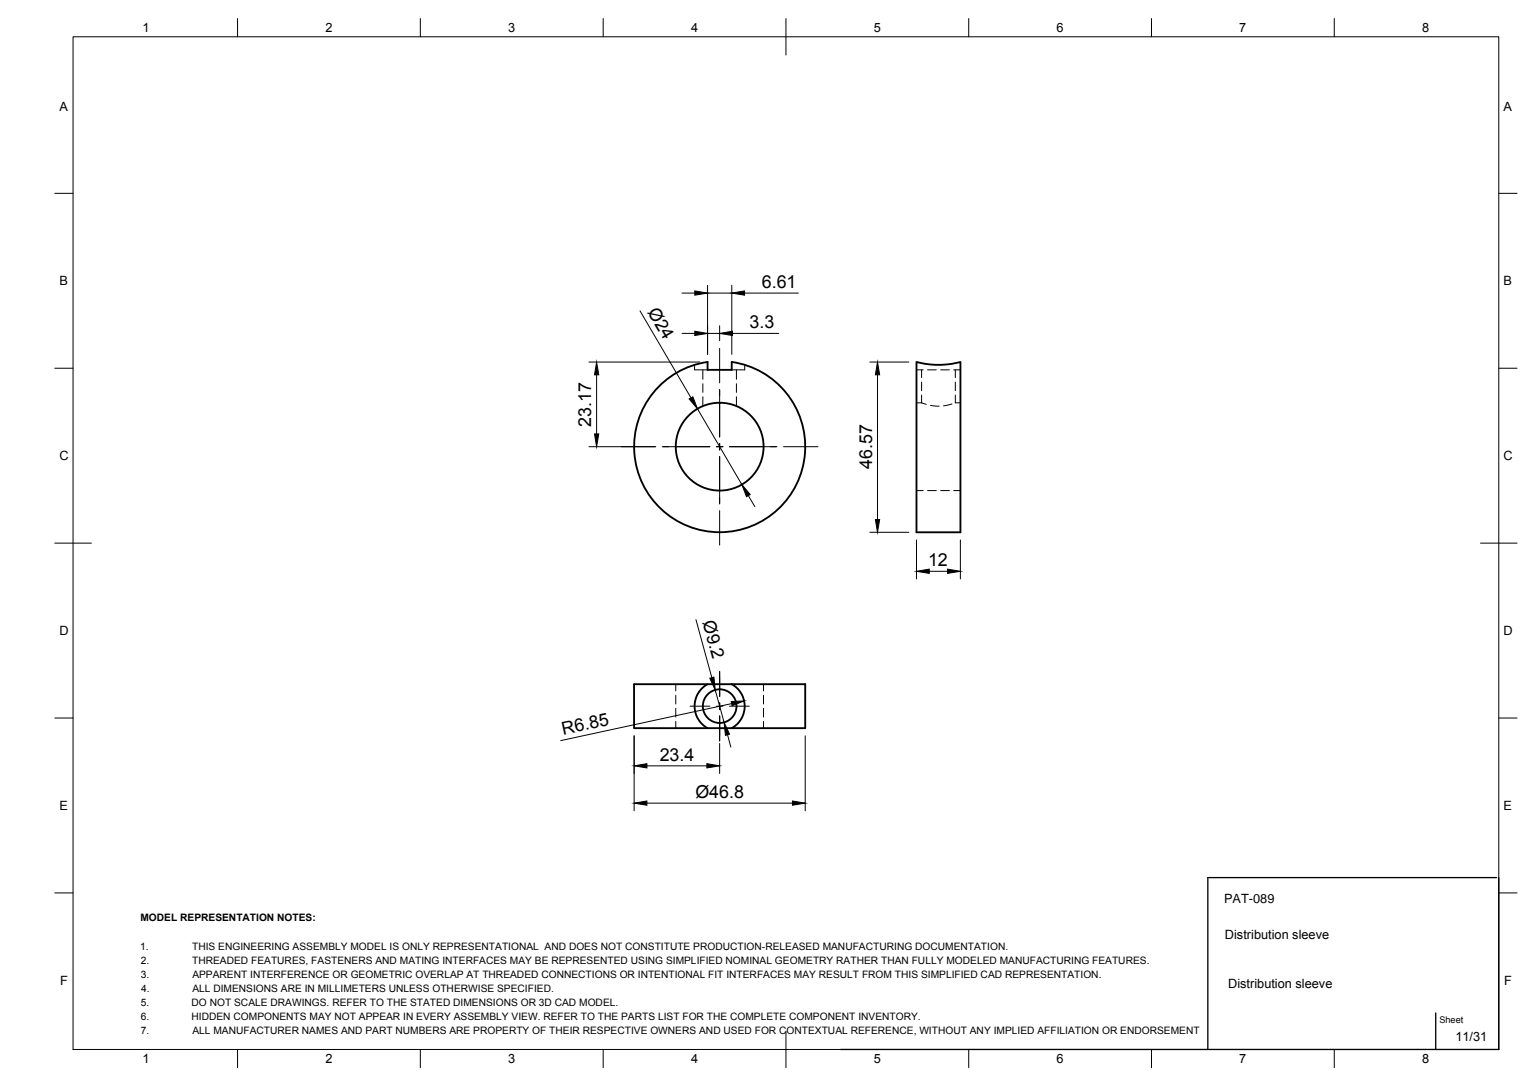
ISO-10303-21;
HEADER;
/* Generated by software containing ST-Developer
 * from STEP Tools, Inc. (www.steptools.com) 
 */

FILE_DESCRIPTION(
/* description */ ('Rotary union on bearing shaft'),
/* implementation_level */ '2;1');

FILE_NAME(
/* name */ 'Distribution sleeve.step',
/* time_stamp */ '2026-10-28T03:24:01-07:00',
/* author */ (''),
/* organization */ (''),
/* preprocessor_version */ 'ST-DEVELOPER v20.2',
/* originating_system */ 'Autodesk Translation Framework v15.17.0.0',
/* authorisation */ '');

FILE_SCHEMA (('AUTOMOTIVE_DESIGN { 1 0 10303 214 3 1 1 }'));
ENDSEC;

DATA;
#10=MECHANICAL_DESIGN_GEOMETRIC_PRESENTATION_REPRESENTATION('',(#319),#9448);
#229=B_SPLINE_CURVE_WITH_KNOTS('',3,(#7786,#7787,#7788,#7789,#7790,#7791,
#7792,#7793,#7794,#7795,#7796,#7797,#7798,#7799,#7800),.UNSPECIFIED.,.F.,
 .F.,(4,2,2,3,2,2,4),(-0.70773137284392,-0.519428793117576,-0.259714396558788,
0.,0.259714396558788,0.519428793117576,0.707731372984028),.UNSPECIFIED.);
#230=B_SPLINE_CURVE_WITH_KNOTS('',3,(#7812,#7813,#7814,#7815,#7816,#7817,
#7818,#7819,#7820,#7821,#7822,#7823,#7824,#7825),.UNSPECIFIED.,.F.,.F.,
(4,2,2,2,2,2,4),(1.36970442594422,1.55800700581067,1.81772140236946,2.07743579892825,
2.33715019548703,2.59686459204582,2.78516717191228),.UNSPECIFIED.);
#231=B_SPLINE_CURVE_WITH_KNOTS('',3,(#7840,#7841,#7842,#7843,#7844,#7845,
#7846,#7847,#7848,#7849,#7850,#7851,#7852,#7853,#7854,#7855,#7856,#7857),
 .UNSPECIFIED.,.F.,.F.,(4,2,2,2,2,2,2,2,4),(0.,0.175311710953118,0.350623421906236,
0.525787580035871,0.700951738165507,0.876115896295143,1.05128005442478,
1.2265917653779,1.40190347633101),.UNSPECIFIED.);
#232=B_SPLINE_CURVE_WITH_KNOTS('',3,(#7858,#7859,#7860,#7861,#7862,#7863,
#7864,#7865,#7866,#7867,#7868,#7869,#7870,#7871,#7872,#7873,#7874,#7875),
 .UNSPECIFIED.,.F.,.F.,(4,2,2,2,2,2,2,2,4),(1.40190347633101,1.57721518728413,
1.75252689823725,1.92769105636689,2.10285521449652,2.27801937262616,2.45318353075579,
2.62849524170891,2.80380695266203),.UNSPECIFIED.);
#265=SHAPE_REPRESENTATION_RELATIONSHIP('SRR','None',#9565,#292);
#292=ADVANCED_BREP_SHAPE_REPRESENTATION('',(#354),#9425);
#319=STYLED_ITEM('',(#9764),#354);
#354=MANIFOLD_SOLID_BREP('Body1',#4874);
#418=FACE_BOUND('',#1067,.T.);
#419=FACE_BOUND('',#1069,.T.);
#420=FACE_BOUND('',#1073,.T.);
#421=FACE_BOUND('',#1075,.T.);
#529=PLANE('',#5352);
#530=PLANE('',#5354);
#531=PLANE('',#5362);
#727=FACE_OUTER_BOUND('',#1064,.T.);
#728=FACE_OUTER_BOUND('',#1065,.T.);
#729=FACE_OUTER_BOUND('',#1066,.T.);
#730=FACE_OUTER_BOUND('',#1068,.T.);
#731=FACE_OUTER_BOUND('',#1070,.T.);
#732=FACE_OUTER_BOUND('',#1071,.T.);
#733=FACE_OUTER_BOUND('',#1072,.T.);
#734=FACE_OUTER_BOUND('',#1074,.T.);
#1064=EDGE_LOOP('',(#3553,#3554,#3555,#3556));
#1065=EDGE_LOOP('',(#3557,#3558,#3559,#3560));
#1066=EDGE_LOOP('',(#3561,#3562,#3563,#3564));
#1067=EDGE_LOOP('',(#3565));
#1068=EDGE_LOOP('',(#3566,#3567,#3568,#3569));
#1069=EDGE_LOOP('',(#3570));
#1070=EDGE_LOOP('',(#3571,#3572,#3573,#3574));
#1071=EDGE_LOOP('',(#3575,#3576,#3577,#3578,#3579));
#1072=EDGE_LOOP('',(#3580,#3581,#3582,#3583));
#1073=EDGE_LOOP('',(#3584,#3585));
#1074=EDGE_LOOP('',(#3586,#3587,#3588,#3589));
#1075=EDGE_LOOP('',(#3590));
#1436=LINE('',#7784,#1756);
#1437=LINE('',#7802,#1757);
#1438=LINE('',#7807,#1758);
#1439=LINE('',#7811,#1759);
#1440=LINE('',#7827,#1760);
#1441=LINE('',#7828,#1761);
#1442=LINE('',#7876,#1762);
#1443=LINE('',#7879,#1763);
#1756=VECTOR('',#6193,1.);
#1757=VECTOR('',#6194,1.);
#1758=VECTOR('',#6199,1.);
#1759=VECTOR('',#6202,1.);
#1760=VECTOR('',#6205,1.);
#1761=VECTOR('',#6206,1.);
#1762=VECTOR('',#6221,0.46);
#1763=VECTOR('',#6224,1.2);
#2065=CIRCLE('',#5349,0.685);
#2066=CIRCLE('',#5351,0.685);
#2067=CIRCLE('',#5353,0.46);
#2068=CIRCLE('',#5355,2.34);
#2069=CIRCLE('',#5356,1.2);
#2070=CIRCLE('',#5358,2.34);
#2071=CIRCLE('',#5361,1.2);
#2347=VERTEX_POINT('',#7782);
#2348=VERTEX_POINT('',#7783);
#2349=VERTEX_POINT('',#7785);
#2350=VERTEX_POINT('',#7801);
#2351=VERTEX_POINT('',#7805);
#2352=VERTEX_POINT('',#7806);
#2353=VERTEX_POINT('',#7808);
#2354=VERTEX_POINT('',#7810);
#2355=VERTEX_POINT('',#7829);
#2356=VERTEX_POINT('',#7833);
#2357=VERTEX_POINT('',#7838);
#2358=VERTEX_POINT('',#7839);
#2359=VERTEX_POINT('',#7878);
#2804=EDGE_CURVE('',#2347,#2348,#1436,.T.);
#2805=EDGE_CURVE('',#2349,#2347,#229,.T.);
#2806=EDGE_CURVE('',#2350,#2349,#1437,.T.);
#2807=EDGE_CURVE('',#2348,#2350,#2065,.T.);
#2808=EDGE_CURVE('',#2351,#2352,#1438,.T.);
#2809=EDGE_CURVE('',#2353,#2351,#2066,.T.);
#2810=EDGE_CURVE('',#2354,#2353,#1439,.T.);
#2811=EDGE_CURVE('',#2352,#2354,#230,.T.);
#2812=EDGE_CURVE('',#2348,#2351,#1440,.T.);
#2813=EDGE_CURVE('',#2353,#2350,#1441,.T.);
#2814=EDGE_CURVE('',#2355,#2355,#2067,.T.);
#2815=EDGE_CURVE('',#2349,#2354,#2068,.T.);
#2816=EDGE_CURVE('',#2356,#2356,#2069,.T.);
#2817=EDGE_CURVE('',#2347,#2352,#2070,.T.);
#2818=EDGE_CURVE('',#2357,#2358,#231,.T.);
#2819=EDGE_CURVE('',#2358,#2357,#232,.T.);
#2820=EDGE_CURVE('',#2358,#2355,#1442,.T.);
#2821=EDGE_CURVE('',#2356,#2359,#1443,.T.);
#2822=EDGE_CURVE('',#2359,#2359,#2071,.T.);
#3553=ORIENTED_EDGE('',*,*,#2804,.F.);
#3554=ORIENTED_EDGE('',*,*,#2805,.F.);
#3555=ORIENTED_EDGE('',*,*,#2806,.F.);
#3556=ORIENTED_EDGE('',*,*,#2807,.F.);
#3557=ORIENTED_EDGE('',*,*,#2808,.F.);
#3558=ORIENTED_EDGE('',*,*,#2809,.F.);
#3559=ORIENTED_EDGE('',*,*,#2810,.F.);
#3560=ORIENTED_EDGE('',*,*,#2811,.F.);
#3561=ORIENTED_EDGE('',*,*,#2812,.F.);
#3562=ORIENTED_EDGE('',*,*,#2807,.T.);
#3563=ORIENTED_EDGE('',*,*,#2813,.F.);
#3564=ORIENTED_EDGE('',*,*,#2809,.T.);
#3565=ORIENTED_EDGE('',*,*,#2814,.F.);
#3566=ORIENTED_EDGE('',*,*,#2810,.T.);
#3567=ORIENTED_EDGE('',*,*,#2813,.T.);
#3568=ORIENTED_EDGE('',*,*,#2806,.T.);
#3569=ORIENTED_EDGE('',*,*,#2815,.T.);
#3570=ORIENTED_EDGE('',*,*,#2816,.T.);
#3571=ORIENTED_EDGE('',*,*,#2811,.T.);
#3572=ORIENTED_EDGE('',*,*,#2815,.F.);
#3573=ORIENTED_EDGE('',*,*,#2805,.T.);
#3574=ORIENTED_EDGE('',*,*,#2817,.T.);
#3575=ORIENTED_EDGE('',*,*,#2818,.F.);
#3576=ORIENTED_EDGE('',*,*,#2819,.F.);
#3577=ORIENTED_EDGE('',*,*,#2820,.T.);
#3578=ORIENTED_EDGE('',*,*,#2814,.T.);
#3579=ORIENTED_EDGE('',*,*,#2820,.F.);
#3580=ORIENTED_EDGE('',*,*,#2816,.F.);
#3581=ORIENTED_EDGE('',*,*,#2821,.T.);
#3582=ORIENTED_EDGE('',*,*,#2822,.T.);
#3583=ORIENTED_EDGE('',*,*,#2821,.F.);
#3584=ORIENTED_EDGE('',*,*,#2818,.T.);
#3585=ORIENTED_EDGE('',*,*,#2819,.T.);
#3586=ORIENTED_EDGE('',*,*,#2808,.T.);
#3587=ORIENTED_EDGE('',*,*,#2817,.F.);
#3588=ORIENTED_EDGE('',*,*,#2804,.T.);
#3589=ORIENTED_EDGE('',*,*,#2812,.T.);
#3590=ORIENTED_EDGE('',*,*,#2822,.F.);
#4506=CYLINDRICAL_SURFACE('',#5348,0.685);
#4507=CYLINDRICAL_SURFACE('',#5350,0.685);
#4508=CYLINDRICAL_SURFACE('',#5357,2.34);
#4509=CYLINDRICAL_SURFACE('',#5359,0.46);
#4510=CYLINDRICAL_SURFACE('',#5360,1.2);
#4640=ADVANCED_FACE('',(#727),#4506,.F.);
#4641=ADVANCED_FACE('',(#728),#4507,.F.);
#4642=ADVANCED_FACE('',(#729,#418),#529,.T.);
#4643=ADVANCED_FACE('',(#730,#419),#530,.T.);
#4644=ADVANCED_FACE('',(#731),#4508,.T.);
#4645=ADVANCED_FACE('',(#732),#4509,.F.);
#4646=ADVANCED_FACE('',(#733,#420),#4510,.F.);
#4647=ADVANCED_FACE('',(#734,#421),#531,.F.);
#4874=CLOSED_SHELL('',(#4640,#4641,#4642,#4643,#4644,#4645,#4646,#4647));
#5347=AXIS2_PLACEMENT_3D('',#7780,#6189,#6190);
#5348=AXIS2_PLACEMENT_3D('',#7781,#6191,#6192);
#5349=AXIS2_PLACEMENT_3D('',#7803,#6195,#6196);
#5350=AXIS2_PLACEMENT_3D('',#7804,#6197,#6198);
#5351=AXIS2_PLACEMENT_3D('',#7809,#6200,#6201);
#5352=AXIS2_PLACEMENT_3D('',#7826,#6203,#6204);
#5353=AXIS2_PLACEMENT_3D('',#7830,#6207,#6208);
#5354=AXIS2_PLACEMENT_3D('',#7831,#6209,#6210);
#5355=AXIS2_PLACEMENT_3D('',#7832,#6211,#6212);
#5356=AXIS2_PLACEMENT_3D('',#7834,#6213,#6214);
#5357=AXIS2_PLACEMENT_3D('',#7835,#6215,#6216);
#5358=AXIS2_PLACEMENT_3D('',#7836,#6217,#6218);
#5359=AXIS2_PLACEMENT_3D('',#7837,#6219,#6220);
#5360=AXIS2_PLACEMENT_3D('',#7877,#6222,#6223);
#5361=AXIS2_PLACEMENT_3D('',#7880,#6225,#6226);
#5362=AXIS2_PLACEMENT_3D('',#7881,#6227,#6228);
#6189=DIRECTION('axis',(0.,0.,1.));
#6190=DIRECTION('refdir',(1.,0.,0.));
#6191=DIRECTION('center_axis',(1.,0.,0.));
#6192=DIRECTION('ref_axis',(0.,0.,-1.));
#6193=DIRECTION('',(-1.,0.,0.));
#6194=DIRECTION('',(1.,0.,0.));
#6195=DIRECTION('center_axis',(1.,0.,0.));
#6196=DIRECTION('ref_axis',(0.,0.,-1.));
#6197=DIRECTION('center_axis',(1.,0.,0.));
#6198=DIRECTION('ref_axis',(0.,7.6571373978539E-16,1.));
#6199=DIRECTION('',(1.,0.,0.));
#6200=DIRECTION('center_axis',(1.,0.,0.));
#6201=DIRECTION('ref_axis',(0.,0.,-1.));
#6202=DIRECTION('',(-1.,0.,0.));
#6203=DIRECTION('center_axis',(1.,0.,0.));
#6204=DIRECTION('ref_axis',(0.,0.,-1.));
#6205=DIRECTION('',(0.,0.,1.));
#6206=DIRECTION('',(0.,0.,-1.));
#6207=DIRECTION('center_axis',(1.,0.,0.));
#6208=DIRECTION('ref_axis',(0.,0.,-1.));
#6209=DIRECTION('center_axis',(0.,1.,0.));
#6210=DIRECTION('ref_axis',(1.,0.,0.));
#6211=DIRECTION('center_axis',(0.,1.,0.));
#6212=DIRECTION('ref_axis',(1.,0.,0.));
#6213=DIRECTION('center_axis',(0.,-1.,0.));
#6214=DIRECTION('ref_axis',(1.,0.,0.));
#6215=DIRECTION('center_axis',(0.,1.,0.));
#6216=DIRECTION('ref_axis',(-1.,0.,1.22464679914735E-16));
#6217=DIRECTION('center_axis',(0.,1.,0.));
#6218=DIRECTION('ref_axis',(1.,0.,0.));
#6219=DIRECTION('center_axis',(1.,0.,0.));
#6220=DIRECTION('ref_axis',(0.,0.,-1.));
#6221=DIRECTION('',(1.,0.,0.));
#6222=DIRECTION('center_axis',(0.,1.,0.));
#6223=DIRECTION('ref_axis',(1.,0.,0.));
#6224=DIRECTION('',(0.,-1.,0.));
#6225=DIRECTION('center_axis',(0.,-1.,0.));
#6226=DIRECTION('ref_axis',(1.,0.,0.));
#6227=DIRECTION('center_axis',(0.,1.,0.));
#6228=DIRECTION('ref_axis',(1.,0.,0.));
#7780=CARTESIAN_POINT('',(0.,0.,0.));
#7781=CARTESIAN_POINT('Origin',(2.1,3.,4.5));
#7782=CARTESIAN_POINT('',(2.3165437617278,2.4,4.16950794260678));
#7783=CARTESIAN_POINT('',(2.1,2.4,4.16950794260678));
#7784=CARTESIAN_POINT('',(2.1,2.4,4.16950794260678));
#7785=CARTESIAN_POINT('',(2.3165437617278,3.6,4.16950794260679));
#7786=CARTESIAN_POINT('Ctrl Pts',(2.3165437617278,3.6,4.16950794260679));
#7787=CARTESIAN_POINT('Ctrl Pts',(2.30831151031136,3.56821604889379,4.11180498050191));
#7788=CARTESIAN_POINT('Ctrl Pts',(2.29860746123388,3.52826296991183,4.05952667968626));
#7789=CARTESIAN_POINT('Ctrl Pts',(2.27651111163957,3.42382665942891,3.95509036920334));
#7790=CARTESIAN_POINT('Ctrl Pts',(2.26271374962431,3.34714352725108,3.90246321020553));
#7791=CARTESIAN_POINT('Ctrl Pts',(2.24304290799559,3.17853989239017,3.83240559410195));
#7792=CARTESIAN_POINT('Ctrl Pts',(2.23749301674888,3.0865714655196,3.815));
#7793=CARTESIAN_POINT('Ctrl Pts',(2.23749301674888,3.,3.815));
#7794=CARTESIAN_POINT('Ctrl Pts',(2.23749301674888,2.9134285344804,3.815));
#7795=CARTESIAN_POINT('Ctrl Pts',(2.24304290799559,2.82146010760983,3.83240559410195));
#7796=CARTESIAN_POINT('Ctrl Pts',(2.26271374962431,2.65285647274892,3.90246321020553));
#7797=CARTESIAN_POINT('Ctrl Pts',(2.27651111163957,2.57617334057109,3.95509036920334));
#7798=CARTESIAN_POINT('Ctrl Pts',(2.29860746124079,2.47173703005551,4.05952667971892));
#7799=CARTESIAN_POINT('Ctrl Pts',(2.30831151030122,2.43178395114536,4.11180498043082));
#7800=CARTESIAN_POINT('Ctrl Pts',(2.3165437617278,2.4,4.16950794260678));
#7801=CARTESIAN_POINT('',(2.1,3.6,4.16950794260679));
#7802=CARTESIAN_POINT('',(2.1,3.6,4.16950794260679));
#7803=CARTESIAN_POINT('Origin',(2.1,3.,4.5));
#7804=CARTESIAN_POINT('Origin',(2.1,3.,4.5));
#7805=CARTESIAN_POINT('',(2.1,2.4,4.83049205739322));
#7806=CARTESIAN_POINT('',(2.3165437617278,2.4,4.83049205739322));
#7807=CARTESIAN_POINT('',(2.1,2.4,4.83049205739322));
#7808=CARTESIAN_POINT('',(2.1,3.6,4.83049205739321));
#7809=CARTESIAN_POINT('Origin',(2.1,3.,4.5));
#7810=CARTESIAN_POINT('',(2.3165437617278,3.6,4.83049205739322));
#7811=CARTESIAN_POINT('',(2.1,3.6,4.83049205739321));
#7812=CARTESIAN_POINT('Ctrl Pts',(2.3165437617278,2.4,4.83049205739322));
#7813=CARTESIAN_POINT('Ctrl Pts',(2.30831151030122,2.43178395114536,4.88819501956918));
#7814=CARTESIAN_POINT('Ctrl Pts',(2.29860746124079,2.47173703005551,4.94047332028108));
#7815=CARTESIAN_POINT('Ctrl Pts',(2.27651111163957,2.57617334057109,5.04490963079666));
#7816=CARTESIAN_POINT('Ctrl Pts',(2.26271374962431,2.65285647274892,5.09753678979447));
#7817=CARTESIAN_POINT('Ctrl Pts',(2.24304290799559,2.82146010760983,5.16759440589805));
#7818=CARTESIAN_POINT('Ctrl Pts',(2.23749301674888,2.9134285344804,5.185));
#7819=CARTESIAN_POINT('Ctrl Pts',(2.23749301674888,3.0865714655196,5.185));
#7820=CARTESIAN_POINT('Ctrl Pts',(2.24304290799559,3.17853989239017,5.16759440589805));
#7821=CARTESIAN_POINT('Ctrl Pts',(2.26271374962431,3.34714352725108,5.09753678979447));
#7822=CARTESIAN_POINT('Ctrl Pts',(2.27651111163957,3.42382665942891,5.04490963079666));
#7823=CARTESIAN_POINT('Ctrl Pts',(2.29860746124079,3.52826296994449,4.94047332028108));
#7824=CARTESIAN_POINT('Ctrl Pts',(2.30831151030122,3.56821604885464,4.88819501956918));
#7825=CARTESIAN_POINT('Ctrl Pts',(2.3165437617278,3.6,4.83049205739322));
#7826=CARTESIAN_POINT('Origin',(2.1,3.,4.5));
#7827=CARTESIAN_POINT('',(2.1,2.4,4.5));
#7828=CARTESIAN_POINT('',(2.1,3.6,4.5));
#7829=CARTESIAN_POINT('',(2.1,3.,4.96));
#7830=CARTESIAN_POINT('Origin',(2.1,3.,4.5));
#7831=CARTESIAN_POINT('Origin',(0.,3.6,4.5));
#7832=CARTESIAN_POINT('Origin',(0.,3.6,4.5));
#7833=CARTESIAN_POINT('',(-1.2,3.6,4.5));
#7834=CARTESIAN_POINT('Origin',(0.,3.6,4.5));
#7835=CARTESIAN_POINT('Origin',(0.,2.4,4.5));
#7836=CARTESIAN_POINT('Origin',(0.,2.4,4.5));
#7837=CARTESIAN_POINT('Origin',(0.,3.,4.5));
#7838=CARTESIAN_POINT('',(1.10833208019979,3.,4.04));
#7839=CARTESIAN_POINT('',(1.10833208019979,3.,4.96));
#7840=CARTESIAN_POINT('Ctrl Pts',(1.10833208019979,3.,4.04));
#7841=CARTESIAN_POINT('Ctrl Pts',(1.10833208019979,3.05843723698437,4.04));
#7842=CARTESIAN_POINT('Ctrl Pts',(1.11344185362589,3.12030150460074,4.05180175367034));
#7843=CARTESIAN_POINT('Ctrl Pts',(1.13126787543157,3.23342404964254,4.09891723731354));
#7844=CARTESIAN_POINT('Ctrl Pts',(1.14366370619736,3.2847433509607,4.13420511226908));
#7845=CARTESIAN_POINT('Ctrl Pts',(1.16647819892242,3.36576077881991,4.21522254012828));
#7846=CARTESIAN_POINT('Ctrl Pts',(1.17846362995473,3.40107463046863,4.26655493783234));
#7847=CARTESIAN_POINT('Ctrl Pts',(1.19532745919784,3.44820985363556,4.37972785158852));
#7848=CARTESIAN_POINT('Ctrl Pts',(1.2,3.46,4.44161194729012));
#7849=CARTESIAN_POINT('Ctrl Pts',(1.2,3.46,4.55838805270988));
#7850=CARTESIAN_POINT('Ctrl Pts',(1.19532745919784,3.44820985363556,4.62027214841148));
#7851=CARTESIAN_POINT('Ctrl Pts',(1.17846362995473,3.40107463046863,4.73344506216766));
#7852=CARTESIAN_POINT('Ctrl Pts',(1.16647819892242,3.36576077881991,4.78477745987172));
#7853=CARTESIAN_POINT('Ctrl Pts',(1.14366370619736,3.2847433509607,4.86579488773092));
#7854=CARTESIAN_POINT('Ctrl Pts',(1.13126787543157,3.23342404964254,4.90108276268646));
#7855=CARTESIAN_POINT('Ctrl Pts',(1.11344185362589,3.12030150460074,4.94819824632966));
#7856=CARTESIAN_POINT('Ctrl Pts',(1.10833208019979,3.05843723698437,4.96));
#7857=CARTESIAN_POINT('Ctrl Pts',(1.10833208019979,3.,4.96));
#7858=CARTESIAN_POINT('Ctrl Pts',(1.10833208019979,3.,4.96));
#7859=CARTESIAN_POINT('Ctrl Pts',(1.10833208019979,2.94156276301563,4.96));
#7860=CARTESIAN_POINT('Ctrl Pts',(1.11344185362589,2.87969849539926,4.94819824632966));
#7861=CARTESIAN_POINT('Ctrl Pts',(1.13126787543157,2.76657595035746,4.90108276268646));
#7862=CARTESIAN_POINT('Ctrl Pts',(1.14366370619736,2.7152566490393,4.86579488773092));
#7863=CARTESIAN_POINT('Ctrl Pts',(1.16647819892242,2.63423922118009,4.78477745987172));
#7864=CARTESIAN_POINT('Ctrl Pts',(1.17846362995473,2.59892536953137,4.73344506216766));
#7865=CARTESIAN_POINT('Ctrl Pts',(1.19532745919784,2.55179014636444,4.62027214841148));
#7866=CARTESIAN_POINT('Ctrl Pts',(1.2,2.54,4.55838805270988));
#7867=CARTESIAN_POINT('Ctrl Pts',(1.2,2.54,4.44161194729012));
#7868=CARTESIAN_POINT('Ctrl Pts',(1.19532745919784,2.55179014636444,4.37972785158852));
#7869=CARTESIAN_POINT('Ctrl Pts',(1.17846362995473,2.59892536953137,4.26655493783234));
#7870=CARTESIAN_POINT('Ctrl Pts',(1.16647819892242,2.63423922118009,4.21522254012828));
#7871=CARTESIAN_POINT('Ctrl Pts',(1.14366370619736,2.7152566490393,4.13420511226908));
#7872=CARTESIAN_POINT('Ctrl Pts',(1.13126787543157,2.76657595035746,4.09891723731354));
#7873=CARTESIAN_POINT('Ctrl Pts',(1.11344185362589,2.87969849539925,4.05180175367034));
#7874=CARTESIAN_POINT('Ctrl Pts',(1.10833208019979,2.94156276301563,4.04));
#7875=CARTESIAN_POINT('Ctrl Pts',(1.10833208019979,3.,4.04));
#7876=CARTESIAN_POINT('',(0.,3.,4.96));
#7877=CARTESIAN_POINT('Origin',(0.,2.4,4.5));
#7878=CARTESIAN_POINT('',(-1.2,2.4,4.5));
#7879=CARTESIAN_POINT('',(-1.2,2.4,4.5));
#7880=CARTESIAN_POINT('Origin',(0.,2.4,4.5));
#7881=CARTESIAN_POINT('Origin',(0.,2.4,4.5));
#9393=UNCERTAINTY_MEASURE_WITH_UNIT(LENGTH_MEASURE(0.001),#9449,
'DISTANCE_ACCURACY_VALUE',
'Maximum model space distance between geometric entities at asserted c
onnectivities');
#9416=UNCERTAINTY_MEASURE_WITH_UNIT(LENGTH_MEASURE(0.001),#9449,
'DISTANCE_ACCURACY_VALUE',
'Maximum model space distance between geometric entities at asserted c
onnectivities');
#9425=(
GEOMETRIC_REPRESENTATION_CONTEXT(3)
GLOBAL_UNCERTAINTY_ASSIGNED_CONTEXT((#9393))
GLOBAL_UNIT_ASSIGNED_CONTEXT((#9449,#9451,#9452))
REPRESENTATION_CONTEXT('','3D')
);
#9448=(
GEOMETRIC_REPRESENTATION_CONTEXT(3)
GLOBAL_UNCERTAINTY_ASSIGNED_CONTEXT((#9416))
GLOBAL_UNIT_ASSIGNED_CONTEXT((#9449,#9451,#9452))
REPRESENTATION_CONTEXT('','3D')
);
#9449=(
LENGTH_UNIT()
NAMED_UNIT(*)
SI_UNIT(.CENTI.,.METRE.)
);
#9451=(
NAMED_UNIT(*)
PLANE_ANGLE_UNIT()
SI_UNIT($,.RADIAN.)
);
#9452=(
NAMED_UNIT(*)
SI_UNIT($,.STERADIAN.)
SOLID_ANGLE_UNIT()
);
#9461=SHAPE_DEFINITION_REPRESENTATION(#9492,#9565);
#9492=PRODUCT_DEFINITION_SHAPE('',$,#9597);
#9565=SHAPE_REPRESENTATION('',(#5347),#9425);
#9588=PRODUCT_DEFINITION_CONTEXT('part definition',#9683,'design');
#9597=PRODUCT_DEFINITION('Distribution sleeve','Distribution sleeve',#9628,
#9588);
#9628=PRODUCT_DEFINITION_FORMATION('',$,#9693);
#9683=APPLICATION_CONTEXT(
'Core Data for Automotive Mechanical Design Process');
#9684=PRODUCT_CONTEXT('part definition',#9683,'mechanical');
#9693=PRODUCT('Distribution sleeve','Distribution sleeve',
'Distribution sleeve',(#9684));
#9758=COLOUR_RGB('Light Blue',0.38,0.62,0.78);
#9759=FILL_AREA_STYLE_COLOUR('',#9758);
#9760=FILL_AREA_STYLE('',(#9759));
#9761=SURFACE_STYLE_FILL_AREA(#9760);
#9762=SURFACE_SIDE_STYLE('',(#9761));
#9763=SURFACE_STYLE_USAGE(.BOTH.,#9762);
#9764=PRESENTATION_STYLE_ASSIGNMENT((#9763));
ENDSEC;
END-ISO-10303-21;
